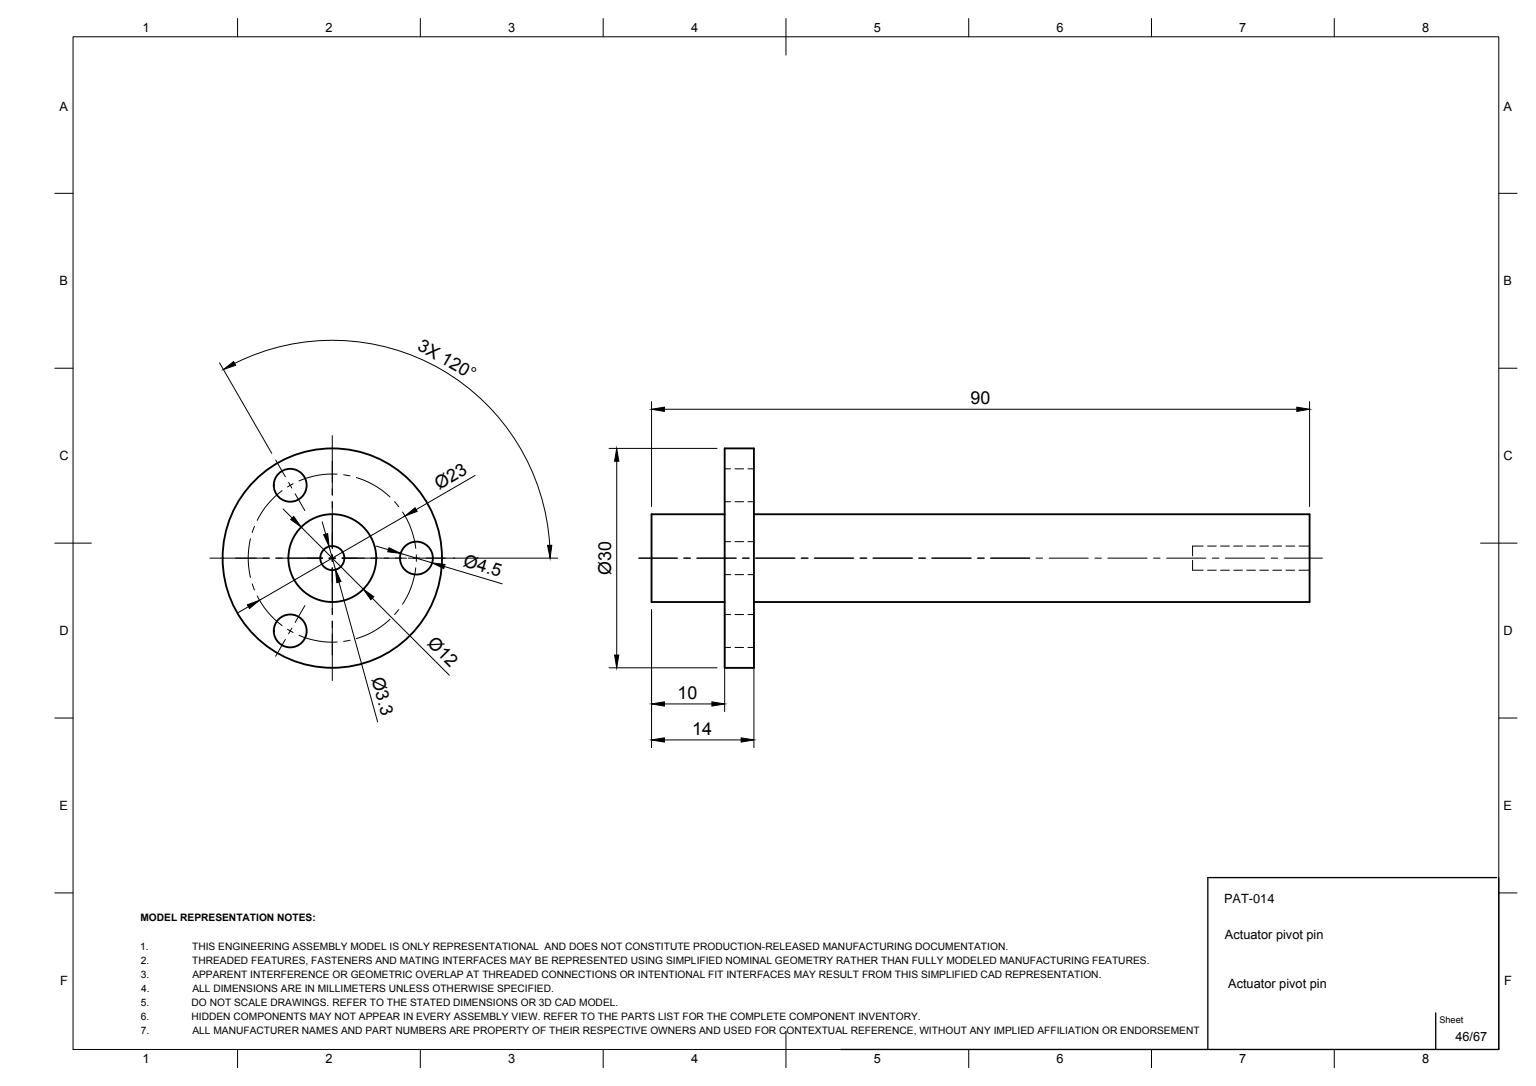
ISO-10303-21;
HEADER;
/* Generated by software containing ST-Developer
 * from STEP Tools, Inc. (www.steptools.com) 
 */

FILE_DESCRIPTION(
/* description */ ('Bin tilter linkage'),
/* implementation_level */ '2;1');

FILE_NAME(
/* name */ 'Actuator pivot pin.step',
/* time_stamp */ '2026-10-28T03:26:24-07:00',
/* author */ (''),
/* organization */ (''),
/* preprocessor_version */ 'ST-DEVELOPER v20.2',
/* originating_system */ 'Autodesk Translation Framework v15.17.0.0',
/* authorisation */ '');

FILE_SCHEMA (('AUTOMOTIVE_DESIGN { 1 0 10303 214 3 1 1 }'));
ENDSEC;

DATA;
#10=MECHANICAL_DESIGN_GEOMETRIC_PRESENTATION_REPRESENTATION('',(#950),#23728);
#730=SHAPE_REPRESENTATION_RELATIONSHIP('SRR','None',#24198,#836);
#836=ADVANCED_BREP_SHAPE_REPRESENTATION('',(#1063),#23698);
#950=STYLED_ITEM('',(#24765),#1063);
#1063=MANIFOLD_SOLID_BREP('Body1',#12481);
#1411=FACE_BOUND('',#3589,.T.);
#1412=FACE_BOUND('',#3590,.T.);
#1413=FACE_BOUND('',#3591,.T.);
#1414=FACE_BOUND('',#3592,.T.);
#1415=FACE_BOUND('',#3594,.T.);
#1416=FACE_BOUND('',#3595,.T.);
#1417=FACE_BOUND('',#3596,.T.);
#1418=FACE_BOUND('',#3597,.T.);
#1419=FACE_BOUND('',#3603,.T.);
#1781=PLANE('',#15016);
#1782=PLANE('',#15026);
#1783=PLANE('',#15029);
#1784=PLANE('',#15037);
#1785=PLANE('',#15038);
#2482=FACE_OUTER_BOUND('',#3583,.T.);
#2483=FACE_OUTER_BOUND('',#3584,.T.);
#2484=FACE_OUTER_BOUND('',#3585,.T.);
#2485=FACE_OUTER_BOUND('',#3586,.T.);
#2486=FACE_OUTER_BOUND('',#3587,.T.);
#2487=FACE_OUTER_BOUND('',#3588,.T.);
#2488=FACE_OUTER_BOUND('',#3593,.T.);
#2489=FACE_OUTER_BOUND('',#3598,.T.);
#2490=FACE_OUTER_BOUND('',#3599,.T.);
#2491=FACE_OUTER_BOUND('',#3600,.T.);
#2492=FACE_OUTER_BOUND('',#3601,.T.);
#2493=FACE_OUTER_BOUND('',#3602,.T.);
#3583=EDGE_LOOP('',(#10597,#10598,#10599,#10600));
#3584=EDGE_LOOP('',(#10601));
#3585=EDGE_LOOP('',(#10602,#10603,#10604,#10605));
#3586=EDGE_LOOP('',(#10606,#10607,#10608,#10609));
#3587=EDGE_LOOP('',(#10610,#10611,#10612,#10613));
#3588=EDGE_LOOP('',(#10614));
#3589=EDGE_LOOP('',(#10615));
#3590=EDGE_LOOP('',(#10616));
#3591=EDGE_LOOP('',(#10617));
#3592=EDGE_LOOP('',(#10618));
#3593=EDGE_LOOP('',(#10619));
#3594=EDGE_LOOP('',(#10620));
#3595=EDGE_LOOP('',(#10621));
#3596=EDGE_LOOP('',(#10622));
#3597=EDGE_LOOP('',(#10623));
#3598=EDGE_LOOP('',(#10624,#10625,#10626,#10627));
#3599=EDGE_LOOP('',(#10628,#10629,#10630,#10631));
#3600=EDGE_LOOP('',(#10632,#10633,#10634,#10635));
#3601=EDGE_LOOP('',(#10636));
#3602=EDGE_LOOP('',(#10637));
#3603=EDGE_LOOP('',(#10638));
#4340=LINE('',#22633,#5015);
#4341=LINE('',#22640,#5016);
#4342=LINE('',#22646,#5017);
#4343=LINE('',#22652,#5018);
#4344=LINE('',#22665,#5019);
#4345=LINE('',#22668,#5020);
#4346=LINE('',#22673,#5021);
#5015=VECTOR('',#18643,0.164999999999999);
#5016=VECTOR('',#18652,0.225);
#5017=VECTOR('',#18659,0.225);
#5018=VECTOR('',#18666,0.225);
#5019=VECTOR('',#18683,1.5);
#5020=VECTOR('',#18686,0.6);
#5021=VECTOR('',#18693,0.6);
#5806=CIRCLE('',#15014,0.164999999999999);
#5807=CIRCLE('',#15015,0.164999999999999);
#5808=CIRCLE('',#15018,0.225);
#5809=CIRCLE('',#15019,0.225);
#5810=CIRCLE('',#15021,0.225);
#5811=CIRCLE('',#15022,0.225);
#5812=CIRCLE('',#15024,0.225);
#5813=CIRCLE('',#15025,0.225);
#5814=CIRCLE('',#15027,1.5);
#5815=CIRCLE('',#15028,0.6);
#5816=CIRCLE('',#15030,1.5);
#5817=CIRCLE('',#15031,0.6);
#5818=CIRCLE('',#15034,0.6);
#5819=CIRCLE('',#15036,0.6);
#6705=VERTEX_POINT('',#22630);
#6706=VERTEX_POINT('',#22632);
#6707=VERTEX_POINT('',#22637);
#6708=VERTEX_POINT('',#22639);
#6709=VERTEX_POINT('',#22643);
#6710=VERTEX_POINT('',#22645);
#6711=VERTEX_POINT('',#22649);
#6712=VERTEX_POINT('',#22651);
#6713=VERTEX_POINT('',#22655);
#6714=VERTEX_POINT('',#22657);
#6715=VERTEX_POINT('',#22660);
#6716=VERTEX_POINT('',#22662);
#6717=VERTEX_POINT('',#22667);
#6718=VERTEX_POINT('',#22671);
#8038=EDGE_CURVE('',#6705,#6705,#5806,.T.);
#8039=EDGE_CURVE('',#6705,#6706,#4340,.T.);
#8040=EDGE_CURVE('',#6706,#6706,#5807,.T.);
#8041=EDGE_CURVE('',#6707,#6707,#5808,.T.);
#8042=EDGE_CURVE('',#6707,#6708,#4341,.T.);
#8043=EDGE_CURVE('',#6708,#6708,#5809,.T.);
#8044=EDGE_CURVE('',#6709,#6709,#5810,.T.);
#8045=EDGE_CURVE('',#6709,#6710,#4342,.T.);
#8046=EDGE_CURVE('',#6710,#6710,#5811,.T.);
#8047=EDGE_CURVE('',#6711,#6711,#5812,.T.);
#8048=EDGE_CURVE('',#6711,#6712,#4343,.T.);
#8049=EDGE_CURVE('',#6712,#6712,#5813,.T.);
#8050=EDGE_CURVE('',#6713,#6713,#5814,.T.);
#8051=EDGE_CURVE('',#6714,#6714,#5815,.T.);
#8052=EDGE_CURVE('',#6715,#6715,#5816,.T.);
#8053=EDGE_CURVE('',#6716,#6716,#5817,.T.);
#8054=EDGE_CURVE('',#6713,#6715,#4344,.T.);
#8055=EDGE_CURVE('',#6716,#6717,#4345,.T.);
#8056=EDGE_CURVE('',#6717,#6717,#5818,.T.);
#8057=EDGE_CURVE('',#6718,#6718,#5819,.T.);
#8058=EDGE_CURVE('',#6718,#6714,#4346,.T.);
#10597=ORIENTED_EDGE('',*,*,#8038,.F.);
#10598=ORIENTED_EDGE('',*,*,#8039,.T.);
#10599=ORIENTED_EDGE('',*,*,#8040,.T.);
#10600=ORIENTED_EDGE('',*,*,#8039,.F.);
#10601=ORIENTED_EDGE('',*,*,#8040,.F.);
#10602=ORIENTED_EDGE('',*,*,#8041,.F.);
#10603=ORIENTED_EDGE('',*,*,#8042,.T.);
#10604=ORIENTED_EDGE('',*,*,#8043,.F.);
#10605=ORIENTED_EDGE('',*,*,#8042,.F.);
#10606=ORIENTED_EDGE('',*,*,#8044,.F.);
#10607=ORIENTED_EDGE('',*,*,#8045,.T.);
#10608=ORIENTED_EDGE('',*,*,#8046,.F.);
#10609=ORIENTED_EDGE('',*,*,#8045,.F.);
#10610=ORIENTED_EDGE('',*,*,#8047,.F.);
#10611=ORIENTED_EDGE('',*,*,#8048,.T.);
#10612=ORIENTED_EDGE('',*,*,#8049,.F.);
#10613=ORIENTED_EDGE('',*,*,#8048,.F.);
#10614=ORIENTED_EDGE('',*,*,#8050,.T.);
#10615=ORIENTED_EDGE('',*,*,#8043,.T.);
#10616=ORIENTED_EDGE('',*,*,#8046,.T.);
#10617=ORIENTED_EDGE('',*,*,#8049,.T.);
#10618=ORIENTED_EDGE('',*,*,#8051,.F.);
#10619=ORIENTED_EDGE('',*,*,#8052,.F.);
#10620=ORIENTED_EDGE('',*,*,#8041,.T.);
#10621=ORIENTED_EDGE('',*,*,#8044,.T.);
#10622=ORIENTED_EDGE('',*,*,#8047,.T.);
#10623=ORIENTED_EDGE('',*,*,#8053,.F.);
#10624=ORIENTED_EDGE('',*,*,#8050,.F.);
#10625=ORIENTED_EDGE('',*,*,#8054,.T.);
#10626=ORIENTED_EDGE('',*,*,#8052,.T.);
#10627=ORIENTED_EDGE('',*,*,#8054,.F.);
#10628=ORIENTED_EDGE('',*,*,#8053,.T.);
#10629=ORIENTED_EDGE('',*,*,#8055,.T.);
#10630=ORIENTED_EDGE('',*,*,#8056,.T.);
#10631=ORIENTED_EDGE('',*,*,#8055,.F.);
#10632=ORIENTED_EDGE('',*,*,#8057,.F.);
#10633=ORIENTED_EDGE('',*,*,#8058,.T.);
#10634=ORIENTED_EDGE('',*,*,#8051,.T.);
#10635=ORIENTED_EDGE('',*,*,#8058,.F.);
#10636=ORIENTED_EDGE('',*,*,#8057,.T.);
#10637=ORIENTED_EDGE('',*,*,#8056,.F.);
#10638=ORIENTED_EDGE('',*,*,#8038,.T.);
#11546=CYLINDRICAL_SURFACE('',#15013,0.164999999999999);
#11547=CYLINDRICAL_SURFACE('',#15017,0.225);
#11548=CYLINDRICAL_SURFACE('',#15020,0.225);
#11549=CYLINDRICAL_SURFACE('',#15023,0.225);
#11550=CYLINDRICAL_SURFACE('',#15032,1.5);
#11551=CYLINDRICAL_SURFACE('',#15033,0.6);
#11552=CYLINDRICAL_SURFACE('',#15035,0.6);
#12207=ADVANCED_FACE('',(#2482),#11546,.F.);
#12208=ADVANCED_FACE('',(#2483),#1781,.F.);
#12209=ADVANCED_FACE('',(#2484),#11547,.F.);
#12210=ADVANCED_FACE('',(#2485),#11548,.F.);
#12211=ADVANCED_FACE('',(#2486),#11549,.F.);
#12212=ADVANCED_FACE('',(#2487,#1411,#1412,#1413,#1414),#1782,.T.);
#12213=ADVANCED_FACE('',(#2488,#1415,#1416,#1417,#1418),#1783,.F.);
#12214=ADVANCED_FACE('',(#2489),#11550,.T.);
#12215=ADVANCED_FACE('',(#2490),#11551,.T.);
#12216=ADVANCED_FACE('',(#2491),#11552,.T.);
#12217=ADVANCED_FACE('',(#2492),#1784,.T.);
#12218=ADVANCED_FACE('',(#2493,#1419),#1785,.F.);
#12481=CLOSED_SHELL('',(#12207,#12208,#12209,#12210,#12211,#12212,#12213,
#12214,#12215,#12216,#12217,#12218));
#15012=AXIS2_PLACEMENT_3D('',#22628,#18637,#18638);
#15013=AXIS2_PLACEMENT_3D('',#22629,#18639,#18640);
#15014=AXIS2_PLACEMENT_3D('',#22631,#18641,#18642);
#15015=AXIS2_PLACEMENT_3D('',#22634,#18644,#18645);
#15016=AXIS2_PLACEMENT_3D('',#22635,#18646,#18647);
#15017=AXIS2_PLACEMENT_3D('',#22636,#18648,#18649);
#15018=AXIS2_PLACEMENT_3D('',#22638,#18650,#18651);
#15019=AXIS2_PLACEMENT_3D('',#22641,#18653,#18654);
#15020=AXIS2_PLACEMENT_3D('',#22642,#18655,#18656);
#15021=AXIS2_PLACEMENT_3D('',#22644,#18657,#18658);
#15022=AXIS2_PLACEMENT_3D('',#22647,#18660,#18661);
#15023=AXIS2_PLACEMENT_3D('',#22648,#18662,#18663);
#15024=AXIS2_PLACEMENT_3D('',#22650,#18664,#18665);
#15025=AXIS2_PLACEMENT_3D('',#22653,#18667,#18668);
#15026=AXIS2_PLACEMENT_3D('',#22654,#18669,#18670);
#15027=AXIS2_PLACEMENT_3D('',#22656,#18671,#18672);
#15028=AXIS2_PLACEMENT_3D('',#22658,#18673,#18674);
#15029=AXIS2_PLACEMENT_3D('',#22659,#18675,#18676);
#15030=AXIS2_PLACEMENT_3D('',#22661,#18677,#18678);
#15031=AXIS2_PLACEMENT_3D('',#22663,#18679,#18680);
#15032=AXIS2_PLACEMENT_3D('',#22664,#18681,#18682);
#15033=AXIS2_PLACEMENT_3D('',#22666,#18684,#18685);
#15034=AXIS2_PLACEMENT_3D('',#22669,#18687,#18688);
#15035=AXIS2_PLACEMENT_3D('',#22670,#18689,#18690);
#15036=AXIS2_PLACEMENT_3D('',#22672,#18691,#18692);
#15037=AXIS2_PLACEMENT_3D('',#22674,#18694,#18695);
#15038=AXIS2_PLACEMENT_3D('',#22675,#18696,#18697);
#18637=DIRECTION('axis',(0.,0.,1.));
#18638=DIRECTION('refdir',(1.,0.,0.));
#18639=DIRECTION('center_axis',(0.,1.,0.));
#18640=DIRECTION('ref_axis',(1.,0.,0.));
#18641=DIRECTION('center_axis',(0.,1.,0.));
#18642=DIRECTION('ref_axis',(1.,0.,0.));
#18643=DIRECTION('',(0.,1.,0.));
#18644=DIRECTION('center_axis',(0.,1.,0.));
#18645=DIRECTION('ref_axis',(1.,0.,0.));
#18646=DIRECTION('center_axis',(0.,1.,0.));
#18647=DIRECTION('ref_axis',(1.,0.,0.));
#18648=DIRECTION('center_axis',(0.,1.,0.));
#18649=DIRECTION('ref_axis',(1.,0.,0.));
#18650=DIRECTION('center_axis',(0.,1.,0.));
#18651=DIRECTION('ref_axis',(1.,0.,0.));
#18652=DIRECTION('',(0.,1.,0.));
#18653=DIRECTION('center_axis',(0.,-1.,0.));
#18654=DIRECTION('ref_axis',(1.,0.,0.));
#18655=DIRECTION('center_axis',(0.,1.,0.));
#18656=DIRECTION('ref_axis',(1.,0.,0.));
#18657=DIRECTION('center_axis',(0.,1.,0.));
#18658=DIRECTION('ref_axis',(1.,0.,0.));
#18659=DIRECTION('',(0.,1.,0.));
#18660=DIRECTION('center_axis',(0.,-1.,0.));
#18661=DIRECTION('ref_axis',(1.,0.,0.));
#18662=DIRECTION('center_axis',(0.,1.,0.));
#18663=DIRECTION('ref_axis',(1.,0.,0.));
#18664=DIRECTION('center_axis',(0.,1.,0.));
#18665=DIRECTION('ref_axis',(1.,0.,0.));
#18666=DIRECTION('',(0.,1.,0.));
#18667=DIRECTION('center_axis',(0.,-1.,0.));
#18668=DIRECTION('ref_axis',(1.,0.,0.));
#18669=DIRECTION('center_axis',(0.,1.,0.));
#18670=DIRECTION('ref_axis',(1.,0.,0.));
#18671=DIRECTION('center_axis',(0.,1.,0.));
#18672=DIRECTION('ref_axis',(1.,0.,0.));
#18673=DIRECTION('center_axis',(0.,1.,0.));
#18674=DIRECTION('ref_axis',(1.,0.,0.));
#18675=DIRECTION('center_axis',(0.,1.,0.));
#18676=DIRECTION('ref_axis',(1.,0.,0.));
#18677=DIRECTION('center_axis',(0.,1.,0.));
#18678=DIRECTION('ref_axis',(1.,0.,0.));
#18679=DIRECTION('center_axis',(0.,-1.,0.));
#18680=DIRECTION('ref_axis',(1.,0.,0.));
#18681=DIRECTION('center_axis',(0.,1.,0.));
#18682=DIRECTION('ref_axis',(1.,0.,0.));
#18683=DIRECTION('',(0.,-1.,0.));
#18684=DIRECTION('center_axis',(0.,1.,0.));
#18685=DIRECTION('ref_axis',(1.,0.,0.));
#18686=DIRECTION('',(0.,-1.,0.));
#18687=DIRECTION('center_axis',(0.,1.,0.));
#18688=DIRECTION('ref_axis',(1.,0.,0.));
#18689=DIRECTION('center_axis',(0.,1.,0.));
#18690=DIRECTION('ref_axis',(1.,0.,0.));
#18691=DIRECTION('center_axis',(0.,1.,0.));
#18692=DIRECTION('ref_axis',(1.,0.,0.));
#18693=DIRECTION('',(0.,-1.,0.));
#18694=DIRECTION('center_axis',(0.,1.,0.));
#18695=DIRECTION('ref_axis',(1.,0.,0.));
#18696=DIRECTION('center_axis',(0.,1.,0.));
#18697=DIRECTION('ref_axis',(1.,0.,0.));
#22628=CARTESIAN_POINT('',(0.,0.,0.));
#22629=CARTESIAN_POINT('Origin',(9.39692620785909,-5.6,18.4202014332567));
#22630=CARTESIAN_POINT('',(9.23192620785909,-5.5,18.4202014332567));
#22631=CARTESIAN_POINT('Origin',(9.39692620785909,-5.5,18.4202014332567));
#22632=CARTESIAN_POINT('',(9.23192620785909,-3.9,18.4202014332567));
#22633=CARTESIAN_POINT('',(9.23192620785909,-5.6,18.4202014332567));
#22634=CARTESIAN_POINT('Origin',(9.39692620785909,-3.9,18.4202014332567));
#22635=CARTESIAN_POINT('Origin',(9.39692620785909,-3.9,18.4202014332567));
#22636=CARTESIAN_POINT('Origin',(10.5469262078591,2.,18.4202014332567));
#22637=CARTESIAN_POINT('',(10.3219262078591,2.1,18.4202014332567));
#22638=CARTESIAN_POINT('Origin',(10.5469262078591,2.1,18.4202014332567));
#22639=CARTESIAN_POINT('',(10.3219262078591,2.5,18.4202014332567));
#22640=CARTESIAN_POINT('',(10.3219262078591,2.,18.4202014332567));
#22641=CARTESIAN_POINT('Origin',(10.5469262078591,2.5,18.4202014332567));
#22642=CARTESIAN_POINT('Origin',(8.82192620785908,2.,19.4161306476088));
#22643=CARTESIAN_POINT('',(8.59692620785908,2.1,19.4161306476088));
#22644=CARTESIAN_POINT('Origin',(8.82192620785908,2.1,19.4161306476088));
#22645=CARTESIAN_POINT('',(8.59692620785908,2.5,19.4161306476088));
#22646=CARTESIAN_POINT('',(8.59692620785908,2.,19.4161306476088));
#22647=CARTESIAN_POINT('Origin',(8.82192620785908,2.5,19.4161306476088));
#22648=CARTESIAN_POINT('Origin',(8.82192620785908,2.,17.4242722189046));
#22649=CARTESIAN_POINT('',(8.59692620785908,2.1,17.4242722189046));
#22650=CARTESIAN_POINT('Origin',(8.82192620785908,2.1,17.4242722189046));
#22651=CARTESIAN_POINT('',(8.59692620785908,2.5,17.4242722189046));
#22652=CARTESIAN_POINT('',(8.59692620785908,2.,17.4242722189046));
#22653=CARTESIAN_POINT('Origin',(8.82192620785908,2.5,17.4242722189046));
#22654=CARTESIAN_POINT('Origin',(9.39692620785909,2.5,18.4202014332567));
#22655=CARTESIAN_POINT('',(7.89692620785909,2.5,18.4202014332567));
#22656=CARTESIAN_POINT('Origin',(9.39692620785909,2.5,18.4202014332567));
#22657=CARTESIAN_POINT('',(8.79692620785909,2.5,18.4202014332567));
#22658=CARTESIAN_POINT('Origin',(9.39692620785909,2.5,18.4202014332567));
#22659=CARTESIAN_POINT('Origin',(9.39692620785909,2.1,18.4202014332567));
#22660=CARTESIAN_POINT('',(7.89692620785909,2.1,18.4202014332567));
#22661=CARTESIAN_POINT('Origin',(9.39692620785909,2.1,18.4202014332567));
#22662=CARTESIAN_POINT('',(8.79692620785909,2.1,18.4202014332567));
#22663=CARTESIAN_POINT('Origin',(9.39692620785909,2.1,18.4202014332567));
#22664=CARTESIAN_POINT('Origin',(9.39692620785909,2.1,18.4202014332567));
#22665=CARTESIAN_POINT('',(7.89692620785909,2.1,18.4202014332567));
#22666=CARTESIAN_POINT('Origin',(9.39692620785909,-5.5,18.4202014332567));
#22667=CARTESIAN_POINT('',(8.79692620785909,-5.5,18.4202014332567));
#22668=CARTESIAN_POINT('',(8.79692620785909,-5.5,18.4202014332567));
#22669=CARTESIAN_POINT('Origin',(9.39692620785909,-5.5,18.4202014332567));
#22670=CARTESIAN_POINT('Origin',(9.39692620785909,-5.5,18.4202014332567));
#22671=CARTESIAN_POINT('',(8.79692620785909,3.5,18.4202014332567));
#22672=CARTESIAN_POINT('Origin',(9.39692620785909,3.5,18.4202014332567));
#22673=CARTESIAN_POINT('',(8.79692620785909,-5.5,18.4202014332567));
#22674=CARTESIAN_POINT('Origin',(9.39692620785909,3.5,18.4202014332567));
#22675=CARTESIAN_POINT('Origin',(9.39692620785909,-5.5,18.4202014332567));
#23581=UNCERTAINTY_MEASURE_WITH_UNIT(LENGTH_MEASURE(0.001),#23729,
'DISTANCE_ACCURACY_VALUE',
'Maximum model space distance between geometric entities at asserted c
onnectivities');
#23611=UNCERTAINTY_MEASURE_WITH_UNIT(LENGTH_MEASURE(0.001),#23729,
'DISTANCE_ACCURACY_VALUE',
'Maximum model space distance between geometric entities at asserted c
onnectivities');
#23698=(
GEOMETRIC_REPRESENTATION_CONTEXT(3)
GLOBAL_UNCERTAINTY_ASSIGNED_CONTEXT((#23581))
GLOBAL_UNIT_ASSIGNED_CONTEXT((#23729,#23731,#23732))
REPRESENTATION_CONTEXT('','3D')
);
#23728=(
GEOMETRIC_REPRESENTATION_CONTEXT(3)
GLOBAL_UNCERTAINTY_ASSIGNED_CONTEXT((#23611))
GLOBAL_UNIT_ASSIGNED_CONTEXT((#23729,#23731,#23732))
REPRESENTATION_CONTEXT('','3D')
);
#23729=(
LENGTH_UNIT()
NAMED_UNIT(*)
SI_UNIT(.CENTI.,.METRE.)
);
#23731=(
NAMED_UNIT(*)
PLANE_ANGLE_UNIT()
SI_UNIT($,.RADIAN.)
);
#23732=(
NAMED_UNIT(*)
SI_UNIT($,.STERADIAN.)
SOLID_ANGLE_UNIT()
);
#23819=SHAPE_DEFINITION_REPRESENTATION(#23986,#24198);
#23986=PRODUCT_DEFINITION_SHAPE('',$,#24315);
#24198=SHAPE_REPRESENTATION('',(#15012),#23698);
#24228=PRODUCT_DEFINITION_CONTEXT('part definition',#24578,'design');
#24315=PRODUCT_DEFINITION('Actuator pivot pin','Actuator pivot pin',#24431,
#24228);
#24431=PRODUCT_DEFINITION_FORMATION('',$,#24666);
#24578=APPLICATION_CONTEXT(
'Core Data for Automotive Mechanical Design Process');
#24579=PRODUCT_CONTEXT('part definition',#24578,'mechanical');
#24666=PRODUCT('Actuator pivot pin','Actuator pivot pin',
'Actuator pivot pin',(#24579));
#24759=COLOUR_RGB('Grey',0.48,0.52,0.57);
#24760=FILL_AREA_STYLE_COLOUR('',#24759);
#24761=FILL_AREA_STYLE('',(#24760));
#24762=SURFACE_STYLE_FILL_AREA(#24761);
#24763=SURFACE_SIDE_STYLE('',(#24762));
#24764=SURFACE_STYLE_USAGE(.BOTH.,#24763);
#24765=PRESENTATION_STYLE_ASSIGNMENT((#24764));
ENDSEC;
END-ISO-10303-21;
